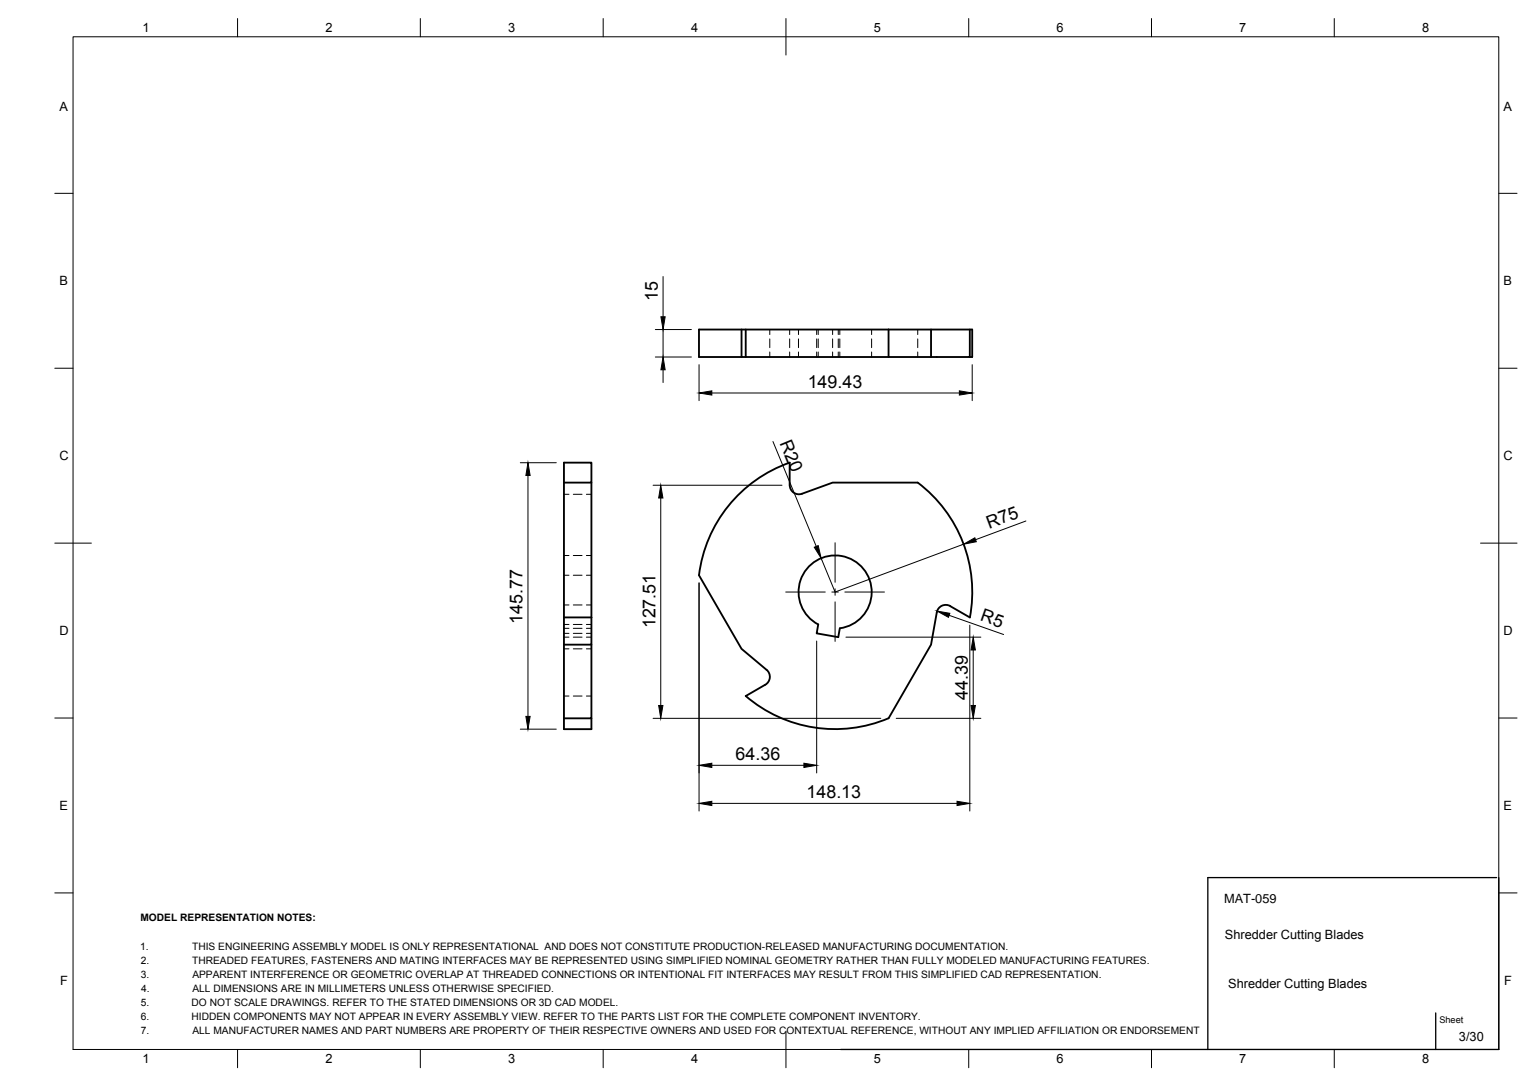
ISO-10303-21;
HEADER;
/* Generated by software containing ST-Developer
 * from STEP Tools, Inc. (www.steptools.com) 
 */

FILE_DESCRIPTION(
/* description */ ('', 'CAx-IF Rec.Pracs.---Representation and Presentation of Product Manufa
cturing Information (PMI)---4.0---2014-10-13'),
/* implementation_level */ '2;1');

FILE_NAME(
/* name */ 'Shredder Cutting Blades.step',
/* time_stamp */ '2026-10-28T23:00:48+01:00',
/* author */ (''),
/* organization */ (''),
/* preprocessor_version */ 'ST-DEVELOPER v20.2',
/* originating_system */ 'Autodesk Translation Framework v15.17.0.0',
/* authorisation */ '');

FILE_SCHEMA (('AP242_MANAGED_MODEL_BASED_3D_ENGINEERING_MIM_LF { 1 0 10303 442 2 1 4 }'));
ENDSEC;

DATA;
#10=MECHANICAL_DESIGN_GEOMETRIC_PRESENTATION_REPRESENTATION('',(#961),#61811);
#911=SHAPE_REPRESENTATION_RELATIONSHIP('SRR','None',#61969,#936);
#936=ADVANCED_BREP_SHAPE_REPRESENTATION('',(#1000),#61782);
#961=STYLED_ITEM('',(#62149),#1000);
#1000=MANIFOLD_SOLID_BREP('Body1',#33791);
#1038=CYLINDRICAL_SURFACE('',#34129,20.);
#1039=CYLINDRICAL_SURFACE('',#34132,5.);
#1040=CYLINDRICAL_SURFACE('',#34137,5.);
#1041=CYLINDRICAL_SURFACE('',#34141,75.);
#1042=CYLINDRICAL_SURFACE('',#34143,75.);
#1043=CYLINDRICAL_SURFACE('',#34145,5.);
#1044=CYLINDRICAL_SURFACE('',#34150,75.);
#1878=FACE_BOUND('',#6114,.T.);
#1879=FACE_BOUND('',#6132,.T.);
#2236=CIRCLE('',#34122,5.);
#2237=CIRCLE('',#34123,75.);
#2238=CIRCLE('',#34124,5.);
#2239=CIRCLE('',#34125,75.);
#2240=CIRCLE('',#34126,5.);
#2241=CIRCLE('',#34127,75.);
#2242=CIRCLE('',#34128,20.);
#2243=CIRCLE('',#34130,20.);
#2244=CIRCLE('',#34133,5.);
#2245=CIRCLE('',#34138,5.);
#2246=CIRCLE('',#34142,75.);
#2247=CIRCLE('',#34144,75.);
#2248=CIRCLE('',#34146,5.);
#2249=CIRCLE('',#34151,75.);
#4232=FACE_OUTER_BOUND('',#6110,.T.);
#4233=FACE_OUTER_BOUND('',#6111,.T.);
#4234=FACE_OUTER_BOUND('',#6112,.T.);
#4235=FACE_OUTER_BOUND('',#6113,.T.);
#4236=FACE_OUTER_BOUND('',#6115,.T.);
#4237=FACE_OUTER_BOUND('',#6116,.T.);
#4238=FACE_OUTER_BOUND('',#6117,.T.);
#4239=FACE_OUTER_BOUND('',#6118,.T.);
#4240=FACE_OUTER_BOUND('',#6119,.T.);
#4241=FACE_OUTER_BOUND('',#6120,.T.);
#4242=FACE_OUTER_BOUND('',#6121,.T.);
#4243=FACE_OUTER_BOUND('',#6122,.T.);
#4244=FACE_OUTER_BOUND('',#6123,.T.);
#4245=FACE_OUTER_BOUND('',#6124,.T.);
#4246=FACE_OUTER_BOUND('',#6125,.T.);
#4247=FACE_OUTER_BOUND('',#6126,.T.);
#4248=FACE_OUTER_BOUND('',#6127,.T.);
#4249=FACE_OUTER_BOUND('',#6128,.T.);
#4250=FACE_OUTER_BOUND('',#6129,.T.);
#4251=FACE_OUTER_BOUND('',#6130,.T.);
#4252=FACE_OUTER_BOUND('',#6131,.T.);
#6110=EDGE_LOOP('',(#21458,#21459,#21460,#21461));
#6111=EDGE_LOOP('',(#21462,#21463,#21464,#21465));
#6112=EDGE_LOOP('',(#21466,#21467,#21468,#21469));
#6113=EDGE_LOOP('',(#21470,#21471,#21472,#21473,#21474,#21475,#21476,#21477,
#21478,#21479,#21480,#21481,#21482,#21483,#21484));
#6114=EDGE_LOOP('',(#21485,#21486,#21487,#21488));
#6115=EDGE_LOOP('',(#21489,#21490,#21491,#21492));
#6116=EDGE_LOOP('',(#21493,#21494,#21495,#21496));
#6117=EDGE_LOOP('',(#21497,#21498,#21499,#21500));
#6118=EDGE_LOOP('',(#21501,#21502,#21503,#21504));
#6119=EDGE_LOOP('',(#21505,#21506,#21507,#21508));
#6120=EDGE_LOOP('',(#21509,#21510,#21511,#21512));
#6121=EDGE_LOOP('',(#21513,#21514,#21515,#21516));
#6122=EDGE_LOOP('',(#21517,#21518,#21519,#21520));
#6123=EDGE_LOOP('',(#21521,#21522,#21523,#21524));
#6124=EDGE_LOOP('',(#21525,#21526,#21527,#21528));
#6125=EDGE_LOOP('',(#21529,#21530,#21531,#21532));
#6126=EDGE_LOOP('',(#21533,#21534,#21535,#21536));
#6127=EDGE_LOOP('',(#21537,#21538,#21539,#21540));
#6128=EDGE_LOOP('',(#21541,#21542,#21543,#21544));
#6129=EDGE_LOOP('',(#21545,#21546,#21547,#21548));
#6130=EDGE_LOOP('',(#21549,#21550,#21551,#21552));
#6131=EDGE_LOOP('',(#21553,#21554,#21555,#21556,#21557,#21558,#21559,#21560,
#21561,#21562,#21563,#21564,#21565,#21566,#21567));
#6132=EDGE_LOOP('',(#21568,#21569,#21570,#21571));
#8346=LINE('',#48842,#10893);
#8347=LINE('',#48844,#10894);
#8348=LINE('',#48846,#10895);
#8349=LINE('',#48847,#10896);
#8350=LINE('',#48851,#10897);
#8351=LINE('',#48853,#10898);
#8352=LINE('',#48855,#10899);
#8353=LINE('',#48856,#10900);
#8354=LINE('',#48858,#10901);
#8355=LINE('',#48859,#10902);
#8356=LINE('',#48863,#10903);
#8357=LINE('',#48865,#10904);
#8358=LINE('',#48869,#10905);
#8359=LINE('',#48873,#10906);
#8360=LINE('',#48875,#10907);
#8361=LINE('',#48879,#10908);
#8362=LINE('',#48883,#10909);
#8363=LINE('',#48885,#10910);
#8364=LINE('',#48889,#10911);
#8365=LINE('',#48896,#10912);
#8366=LINE('',#48898,#10913);
#8367=LINE('',#48899,#10914);
#8368=LINE('',#48902,#10915);
#8369=LINE('',#48906,#10916);
#8370=LINE('',#48907,#10917);
#8371=LINE('',#48910,#10918);
#8372=LINE('',#48911,#10919);
#8373=LINE('',#48914,#10920);
#8374=LINE('',#48916,#10921);
#8375=LINE('',#48917,#10922);
#8376=LINE('',#48920,#10923);
#8377=LINE('',#48924,#10924);
#8378=LINE('',#48925,#10925);
#8379=LINE('',#48928,#10926);
#8380=LINE('',#48929,#10927);
#8381=LINE('',#48933,#10928);
#8382=LINE('',#48938,#10929);
#8383=LINE('',#48941,#10930);
#8384=LINE('',#48944,#10931);
#8385=LINE('',#48945,#10932);
#8386=LINE('',#48947,#10933);
#8387=LINE('',#48950,#10934);
#8388=LINE('',#48951,#10935);
#10893=VECTOR('',#38180,10.);
#10894=VECTOR('',#38181,10.);
#10895=VECTOR('',#38182,10.);
#10896=VECTOR('',#38183,10.);
#10897=VECTOR('',#38186,10.);
#10898=VECTOR('',#38187,10.);
#10899=VECTOR('',#38188,10.);
#10900=VECTOR('',#38189,10.);
#10901=VECTOR('',#38192,9.99999999999999);
#10902=VECTOR('',#38193,9.99999999999999);
#10903=VECTOR('',#38196,10.);
#10904=VECTOR('',#38197,9.99999999999999);
#10905=VECTOR('',#38200,10.);
#10906=VECTOR('',#38203,10.);
#10907=VECTOR('',#38204,10.);
#10908=VECTOR('',#38207,10.);
#10909=VECTOR('',#38210,10.);
#10910=VECTOR('',#38211,10.);
#10911=VECTOR('',#38214,10.);
#10912=VECTOR('',#38225,10.);
#10913=VECTOR('',#38226,10.);
#10914=VECTOR('',#38227,10.);
#10915=VECTOR('',#38230,10.);
#10916=VECTOR('',#38235,10.);
#10917=VECTOR('',#38236,9.99999999999999);
#10918=VECTOR('',#38239,10.);
#10919=VECTOR('',#38240,10.);
#10920=VECTOR('',#38243,10.);
#10921=VECTOR('',#38244,10.);
#10922=VECTOR('',#38245,10.);
#10923=VECTOR('',#38248,10.);
#10924=VECTOR('',#38253,10.);
#10925=VECTOR('',#38254,10.);
#10926=VECTOR('',#38257,10.);
#10927=VECTOR('',#38258,10.);
#10928=VECTOR('',#38263,10.);
#10929=VECTOR('',#38270,10.);
#10930=VECTOR('',#38273,10.);
#10931=VECTOR('',#38276,10.);
#10932=VECTOR('',#38277,10.);
#10933=VECTOR('',#38280,10.);
#10934=VECTOR('',#38283,10.);
#10935=VECTOR('',#38284,10.);
#13440=VERTEX_POINT('',#48840);
#13441=VERTEX_POINT('',#48841);
#13442=VERTEX_POINT('',#48843);
#13443=VERTEX_POINT('',#48845);
#13444=VERTEX_POINT('',#48849);
#13445=VERTEX_POINT('',#48850);
#13446=VERTEX_POINT('',#48852);
#13447=VERTEX_POINT('',#48854);
#13448=VERTEX_POINT('',#48861);
#13449=VERTEX_POINT('',#48862);
#13450=VERTEX_POINT('',#48864);
#13451=VERTEX_POINT('',#48866);
#13452=VERTEX_POINT('',#48868);
#13453=VERTEX_POINT('',#48870);
#13454=VERTEX_POINT('',#48872);
#13455=VERTEX_POINT('',#48874);
#13456=VERTEX_POINT('',#48876);
#13457=VERTEX_POINT('',#48878);
#13458=VERTEX_POINT('',#48880);
#13459=VERTEX_POINT('',#48882);
#13460=VERTEX_POINT('',#48884);
#13461=VERTEX_POINT('',#48886);
#13462=VERTEX_POINT('',#48888);
#13463=VERTEX_POINT('',#48895);
#13464=VERTEX_POINT('',#48897);
#13465=VERTEX_POINT('',#48901);
#13466=VERTEX_POINT('',#48905);
#13467=VERTEX_POINT('',#48909);
#13468=VERTEX_POINT('',#48913);
#13469=VERTEX_POINT('',#48915);
#13470=VERTEX_POINT('',#48919);
#13471=VERTEX_POINT('',#48923);
#13472=VERTEX_POINT('',#48927);
#13473=VERTEX_POINT('',#48931);
#13474=VERTEX_POINT('',#48937);
#13475=VERTEX_POINT('',#48939);
#13476=VERTEX_POINT('',#48943);
#13477=VERTEX_POINT('',#48949);
#16631=EDGE_CURVE('',#13440,#13441,#8346,.T.);
#16632=EDGE_CURVE('',#13440,#13442,#8347,.T.);
#16633=EDGE_CURVE('',#13443,#13442,#8348,.T.);
#16634=EDGE_CURVE('',#13441,#13443,#8349,.T.);
#16635=EDGE_CURVE('',#13444,#13445,#8350,.T.);
#16636=EDGE_CURVE('',#13446,#13444,#8351,.T.);
#16637=EDGE_CURVE('',#13447,#13446,#8352,.T.);
#16638=EDGE_CURVE('',#13445,#13447,#8353,.T.);
#16639=EDGE_CURVE('',#13445,#13440,#8354,.T.);
#16640=EDGE_CURVE('',#13442,#13447,#8355,.T.);
#16641=EDGE_CURVE('',#13448,#13449,#8356,.T.);
#16642=EDGE_CURVE('',#13449,#13450,#8357,.T.);
#16643=EDGE_CURVE('',#13450,#13451,#2236,.T.);
#16644=EDGE_CURVE('',#13451,#13452,#8358,.T.);
#16645=EDGE_CURVE('',#13453,#13452,#2237,.T.);
#16646=EDGE_CURVE('',#13453,#13454,#8359,.T.);
#16647=EDGE_CURVE('',#13454,#13455,#8360,.T.);
#16648=EDGE_CURVE('',#13455,#13456,#2238,.T.);
#16649=EDGE_CURVE('',#13456,#13457,#8361,.T.);
#16650=EDGE_CURVE('',#13458,#13457,#2239,.T.);
#16651=EDGE_CURVE('',#13458,#13459,#8362,.T.);
#16652=EDGE_CURVE('',#13459,#13460,#8363,.T.);
#16653=EDGE_CURVE('',#13460,#13461,#2240,.T.);
#16654=EDGE_CURVE('',#13461,#13462,#8364,.T.);
#16655=EDGE_CURVE('',#13448,#13462,#2241,.T.);
#16656=EDGE_CURVE('',#13446,#13443,#2242,.T.);
#16657=EDGE_CURVE('',#13441,#13444,#2243,.T.);
#16658=EDGE_CURVE('',#13452,#13463,#8365,.T.);
#16659=EDGE_CURVE('',#13451,#13464,#8366,.T.);
#16660=EDGE_CURVE('',#13463,#13464,#8367,.T.);
#16661=EDGE_CURVE('',#13450,#13465,#8368,.T.);
#16662=EDGE_CURVE('',#13464,#13465,#2244,.T.);
#16663=EDGE_CURVE('',#13449,#13466,#8369,.T.);
#16664=EDGE_CURVE('',#13465,#13466,#8370,.T.);
#16665=EDGE_CURVE('',#13467,#13448,#8371,.T.);
#16666=EDGE_CURVE('',#13466,#13467,#8372,.T.);
#16667=EDGE_CURVE('',#13457,#13468,#8373,.T.);
#16668=EDGE_CURVE('',#13456,#13469,#8374,.T.);
#16669=EDGE_CURVE('',#13468,#13469,#8375,.T.);
#16670=EDGE_CURVE('',#13455,#13470,#8376,.T.);
#16671=EDGE_CURVE('',#13469,#13470,#2245,.T.);
#16672=EDGE_CURVE('',#13454,#13471,#8377,.T.);
#16673=EDGE_CURVE('',#13470,#13471,#8378,.T.);
#16674=EDGE_CURVE('',#13472,#13453,#8379,.T.);
#16675=EDGE_CURVE('',#13471,#13472,#8380,.T.);
#16676=EDGE_CURVE('',#13473,#13468,#2246,.T.);
#16677=EDGE_CURVE('',#13473,#13458,#8381,.T.);
#16678=EDGE_CURVE('',#13472,#13463,#2247,.T.);
#16679=EDGE_CURVE('',#13460,#13474,#8382,.T.);
#16680=EDGE_CURVE('',#13475,#13474,#2248,.T.);
#16681=EDGE_CURVE('',#13461,#13475,#8383,.T.);
#16682=EDGE_CURVE('',#13459,#13476,#8384,.T.);
#16683=EDGE_CURVE('',#13474,#13476,#8385,.T.);
#16684=EDGE_CURVE('',#13476,#13473,#8386,.T.);
#16685=EDGE_CURVE('',#13462,#13477,#8387,.T.);
#16686=EDGE_CURVE('',#13477,#13475,#8388,.T.);
#16687=EDGE_CURVE('',#13467,#13477,#2249,.T.);
#21458=ORIENTED_EDGE('',*,*,#16631,.F.);
#21459=ORIENTED_EDGE('',*,*,#16632,.T.);
#21460=ORIENTED_EDGE('',*,*,#16633,.F.);
#21461=ORIENTED_EDGE('',*,*,#16634,.F.);
#21462=ORIENTED_EDGE('',*,*,#16635,.F.);
#21463=ORIENTED_EDGE('',*,*,#16636,.F.);
#21464=ORIENTED_EDGE('',*,*,#16637,.F.);
#21465=ORIENTED_EDGE('',*,*,#16638,.F.);
#21466=ORIENTED_EDGE('',*,*,#16639,.F.);
#21467=ORIENTED_EDGE('',*,*,#16638,.T.);
#21468=ORIENTED_EDGE('',*,*,#16640,.F.);
#21469=ORIENTED_EDGE('',*,*,#16632,.F.);
#21470=ORIENTED_EDGE('',*,*,#16641,.T.);
#21471=ORIENTED_EDGE('',*,*,#16642,.T.);
#21472=ORIENTED_EDGE('',*,*,#16643,.T.);
#21473=ORIENTED_EDGE('',*,*,#16644,.T.);
#21474=ORIENTED_EDGE('',*,*,#16645,.F.);
#21475=ORIENTED_EDGE('',*,*,#16646,.T.);
#21476=ORIENTED_EDGE('',*,*,#16647,.T.);
#21477=ORIENTED_EDGE('',*,*,#16648,.T.);
#21478=ORIENTED_EDGE('',*,*,#16649,.T.);
#21479=ORIENTED_EDGE('',*,*,#16650,.F.);
#21480=ORIENTED_EDGE('',*,*,#16651,.T.);
#21481=ORIENTED_EDGE('',*,*,#16652,.T.);
#21482=ORIENTED_EDGE('',*,*,#16653,.T.);
#21483=ORIENTED_EDGE('',*,*,#16654,.T.);
#21484=ORIENTED_EDGE('',*,*,#16655,.F.);
#21485=ORIENTED_EDGE('',*,*,#16633,.T.);
#21486=ORIENTED_EDGE('',*,*,#16640,.T.);
#21487=ORIENTED_EDGE('',*,*,#16637,.T.);
#21488=ORIENTED_EDGE('',*,*,#16656,.T.);
#21489=ORIENTED_EDGE('',*,*,#16634,.T.);
#21490=ORIENTED_EDGE('',*,*,#16656,.F.);
#21491=ORIENTED_EDGE('',*,*,#16636,.T.);
#21492=ORIENTED_EDGE('',*,*,#16657,.F.);
#21493=ORIENTED_EDGE('',*,*,#16658,.F.);
#21494=ORIENTED_EDGE('',*,*,#16644,.F.);
#21495=ORIENTED_EDGE('',*,*,#16659,.T.);
#21496=ORIENTED_EDGE('',*,*,#16660,.F.);
#21497=ORIENTED_EDGE('',*,*,#16643,.F.);
#21498=ORIENTED_EDGE('',*,*,#16661,.T.);
#21499=ORIENTED_EDGE('',*,*,#16662,.F.);
#21500=ORIENTED_EDGE('',*,*,#16659,.F.);
#21501=ORIENTED_EDGE('',*,*,#16642,.F.);
#21502=ORIENTED_EDGE('',*,*,#16663,.T.);
#21503=ORIENTED_EDGE('',*,*,#16664,.F.);
#21504=ORIENTED_EDGE('',*,*,#16661,.F.);
#21505=ORIENTED_EDGE('',*,*,#16665,.F.);
#21506=ORIENTED_EDGE('',*,*,#16666,.F.);
#21507=ORIENTED_EDGE('',*,*,#16663,.F.);
#21508=ORIENTED_EDGE('',*,*,#16641,.F.);
#21509=ORIENTED_EDGE('',*,*,#16667,.F.);
#21510=ORIENTED_EDGE('',*,*,#16649,.F.);
#21511=ORIENTED_EDGE('',*,*,#16668,.T.);
#21512=ORIENTED_EDGE('',*,*,#16669,.F.);
#21513=ORIENTED_EDGE('',*,*,#16648,.F.);
#21514=ORIENTED_EDGE('',*,*,#16670,.T.);
#21515=ORIENTED_EDGE('',*,*,#16671,.F.);
#21516=ORIENTED_EDGE('',*,*,#16668,.F.);
#21517=ORIENTED_EDGE('',*,*,#16647,.F.);
#21518=ORIENTED_EDGE('',*,*,#16672,.T.);
#21519=ORIENTED_EDGE('',*,*,#16673,.F.);
#21520=ORIENTED_EDGE('',*,*,#16670,.F.);
#21521=ORIENTED_EDGE('',*,*,#16674,.F.);
#21522=ORIENTED_EDGE('',*,*,#16675,.F.);
#21523=ORIENTED_EDGE('',*,*,#16672,.F.);
#21524=ORIENTED_EDGE('',*,*,#16646,.F.);
#21525=ORIENTED_EDGE('',*,*,#16667,.T.);
#21526=ORIENTED_EDGE('',*,*,#16676,.F.);
#21527=ORIENTED_EDGE('',*,*,#16677,.T.);
#21528=ORIENTED_EDGE('',*,*,#16650,.T.);
#21529=ORIENTED_EDGE('',*,*,#16658,.T.);
#21530=ORIENTED_EDGE('',*,*,#16678,.F.);
#21531=ORIENTED_EDGE('',*,*,#16674,.T.);
#21532=ORIENTED_EDGE('',*,*,#16645,.T.);
#21533=ORIENTED_EDGE('',*,*,#16653,.F.);
#21534=ORIENTED_EDGE('',*,*,#16679,.T.);
#21535=ORIENTED_EDGE('',*,*,#16680,.F.);
#21536=ORIENTED_EDGE('',*,*,#16681,.F.);
#21537=ORIENTED_EDGE('',*,*,#16652,.F.);
#21538=ORIENTED_EDGE('',*,*,#16682,.T.);
#21539=ORIENTED_EDGE('',*,*,#16683,.F.);
#21540=ORIENTED_EDGE('',*,*,#16679,.F.);
#21541=ORIENTED_EDGE('',*,*,#16677,.F.);
#21542=ORIENTED_EDGE('',*,*,#16684,.F.);
#21543=ORIENTED_EDGE('',*,*,#16682,.F.);
#21544=ORIENTED_EDGE('',*,*,#16651,.F.);
#21545=ORIENTED_EDGE('',*,*,#16685,.F.);
#21546=ORIENTED_EDGE('',*,*,#16654,.F.);
#21547=ORIENTED_EDGE('',*,*,#16681,.T.);
#21548=ORIENTED_EDGE('',*,*,#16686,.F.);
#21549=ORIENTED_EDGE('',*,*,#16665,.T.);
#21550=ORIENTED_EDGE('',*,*,#16655,.T.);
#21551=ORIENTED_EDGE('',*,*,#16685,.T.);
#21552=ORIENTED_EDGE('',*,*,#16687,.F.);
#21553=ORIENTED_EDGE('',*,*,#16666,.T.);
#21554=ORIENTED_EDGE('',*,*,#16687,.T.);
#21555=ORIENTED_EDGE('',*,*,#16686,.T.);
#21556=ORIENTED_EDGE('',*,*,#16680,.T.);
#21557=ORIENTED_EDGE('',*,*,#16683,.T.);
#21558=ORIENTED_EDGE('',*,*,#16684,.T.);
#21559=ORIENTED_EDGE('',*,*,#16676,.T.);
#21560=ORIENTED_EDGE('',*,*,#16669,.T.);
#21561=ORIENTED_EDGE('',*,*,#16671,.T.);
#21562=ORIENTED_EDGE('',*,*,#16673,.T.);
#21563=ORIENTED_EDGE('',*,*,#16675,.T.);
#21564=ORIENTED_EDGE('',*,*,#16678,.T.);
#21565=ORIENTED_EDGE('',*,*,#16660,.T.);
#21566=ORIENTED_EDGE('',*,*,#16662,.T.);
#21567=ORIENTED_EDGE('',*,*,#16664,.T.);
#21568=ORIENTED_EDGE('',*,*,#16631,.T.);
#21569=ORIENTED_EDGE('',*,*,#16657,.T.);
#21570=ORIENTED_EDGE('',*,*,#16635,.T.);
#21571=ORIENTED_EDGE('',*,*,#16639,.T.);
#31112=PLANE('',#34118);
#31113=PLANE('',#34119);
#31114=PLANE('',#34120);
#31115=PLANE('',#34121);
#31116=PLANE('',#34131);
#31117=PLANE('',#34134);
#31118=PLANE('',#34135);
#31119=PLANE('',#34136);
#31120=PLANE('',#34139);
#31121=PLANE('',#34140);
#31122=PLANE('',#34147);
#31123=PLANE('',#34148);
#31124=PLANE('',#34149);
#31125=PLANE('',#34152);
#31913=ADVANCED_FACE('',(#4232),#31112,.F.);
#31914=ADVANCED_FACE('',(#4233),#31113,.F.);
#31915=ADVANCED_FACE('',(#4234),#31114,.F.);
#31916=ADVANCED_FACE('',(#4235,#1878),#31115,.F.);
#31917=ADVANCED_FACE('',(#4236),#1038,.F.);
#31918=ADVANCED_FACE('',(#4237),#31116,.F.);
#31919=ADVANCED_FACE('',(#4238),#1039,.F.);
#31920=ADVANCED_FACE('',(#4239),#31117,.F.);
#31921=ADVANCED_FACE('',(#4240),#31118,.F.);
#31922=ADVANCED_FACE('',(#4241),#31119,.F.);
#31923=ADVANCED_FACE('',(#4242),#1040,.F.);
#31924=ADVANCED_FACE('',(#4243),#31120,.F.);
#31925=ADVANCED_FACE('',(#4244),#31121,.F.);
#31926=ADVANCED_FACE('',(#4245),#1041,.T.);
#31927=ADVANCED_FACE('',(#4246),#1042,.T.);
#31928=ADVANCED_FACE('',(#4247),#1043,.F.);
#31929=ADVANCED_FACE('',(#4248),#31122,.F.);
#31930=ADVANCED_FACE('',(#4249),#31123,.F.);
#31931=ADVANCED_FACE('',(#4250),#31124,.F.);
#31932=ADVANCED_FACE('',(#4251),#1044,.T.);
#31933=ADVANCED_FACE('',(#4252,#1879),#31125,.T.);
#33791=CLOSED_SHELL('',(#31913,#31914,#31915,#31916,#31917,#31918,#31919,
#31920,#31921,#31922,#31923,#31924,#31925,#31926,#31927,#31928,#31929,#31930,
#31931,#31932,#31933));
#34117=AXIS2_PLACEMENT_3D('',#48838,#38176,#38177);
#34118=AXIS2_PLACEMENT_3D('',#48839,#38178,#38179);
#34119=AXIS2_PLACEMENT_3D('',#48848,#38184,#38185);
#34120=AXIS2_PLACEMENT_3D('',#48857,#38190,#38191);
#34121=AXIS2_PLACEMENT_3D('',#48860,#38194,#38195);
#34122=AXIS2_PLACEMENT_3D('',#48867,#38198,#38199);
#34123=AXIS2_PLACEMENT_3D('',#48871,#38201,#38202);
#34124=AXIS2_PLACEMENT_3D('',#48877,#38205,#38206);
#34125=AXIS2_PLACEMENT_3D('',#48881,#38208,#38209);
#34126=AXIS2_PLACEMENT_3D('',#48887,#38212,#38213);
#34127=AXIS2_PLACEMENT_3D('',#48890,#38215,#38216);
#34128=AXIS2_PLACEMENT_3D('',#48891,#38217,#38218);
#34129=AXIS2_PLACEMENT_3D('',#48892,#38219,#38220);
#34130=AXIS2_PLACEMENT_3D('',#48893,#38221,#38222);
#34131=AXIS2_PLACEMENT_3D('',#48894,#38223,#38224);
#34132=AXIS2_PLACEMENT_3D('',#48900,#38228,#38229);
#34133=AXIS2_PLACEMENT_3D('',#48903,#38231,#38232);
#34134=AXIS2_PLACEMENT_3D('',#48904,#38233,#38234);
#34135=AXIS2_PLACEMENT_3D('',#48908,#38237,#38238);
#34136=AXIS2_PLACEMENT_3D('',#48912,#38241,#38242);
#34137=AXIS2_PLACEMENT_3D('',#48918,#38246,#38247);
#34138=AXIS2_PLACEMENT_3D('',#48921,#38249,#38250);
#34139=AXIS2_PLACEMENT_3D('',#48922,#38251,#38252);
#34140=AXIS2_PLACEMENT_3D('',#48926,#38255,#38256);
#34141=AXIS2_PLACEMENT_3D('',#48930,#38259,#38260);
#34142=AXIS2_PLACEMENT_3D('',#48932,#38261,#38262);
#34143=AXIS2_PLACEMENT_3D('',#48934,#38264,#38265);
#34144=AXIS2_PLACEMENT_3D('',#48935,#38266,#38267);
#34145=AXIS2_PLACEMENT_3D('',#48936,#38268,#38269);
#34146=AXIS2_PLACEMENT_3D('',#48940,#38271,#38272);
#34147=AXIS2_PLACEMENT_3D('',#48942,#38274,#38275);
#34148=AXIS2_PLACEMENT_3D('',#48946,#38278,#38279);
#34149=AXIS2_PLACEMENT_3D('',#48948,#38281,#38282);
#34150=AXIS2_PLACEMENT_3D('',#48952,#38285,#38286);
#34151=AXIS2_PLACEMENT_3D('',#48953,#38287,#38288);
#34152=AXIS2_PLACEMENT_3D('',#48954,#38289,#38290);
#38176=DIRECTION('axis',(0.,0.,1.));
#38177=DIRECTION('refdir',(1.,0.,0.));
#38178=DIRECTION('center_axis',(0.996957691137886,-6.79465961587148E-16,
0.077944609056791));
#38179=DIRECTION('ref_axis',(0.077944609056791,2.83369376080442E-15,-0.996957691137886));
#38180=DIRECTION('',(-0.077944609056791,-2.83369376080442E-15,0.996957691137886));
#38181=DIRECTION('',(-4.56527663898138E-16,-1.,-2.87803349790671E-15));
#38182=DIRECTION('',(0.077944609056791,2.83369376080442E-15,-0.996957691137886));
#38183=DIRECTION('',(-4.56527663898138E-16,-1.,-2.87803349790671E-15));
#38184=DIRECTION('center_axis',(-0.996957691137886,6.79465961587148E-16,
-0.077944609056791));
#38185=DIRECTION('ref_axis',(-0.077944609056791,-2.83369376080442E-15,0.996957691137886));
#38186=DIRECTION('',(0.077944609056791,2.83369376080442E-15,-0.996957691137886));
#38187=DIRECTION('',(4.56527663898138E-16,1.,2.87803349790671E-15));
#38188=DIRECTION('',(-0.077944609056791,-2.83369376080442E-15,0.996957691137886));
#38189=DIRECTION('',(-4.56527663898138E-16,-1.,-2.87803349790671E-15));
#38190=DIRECTION('center_axis',(0.0779446090567893,2.83369376080442E-15,
-0.996957691137886));
#38191=DIRECTION('ref_axis',(-0.996957691137886,6.79465961587143E-16,-0.0779446090567894));
#38192=DIRECTION('',(0.996957691137886,-6.79465961587143E-16,0.0779446090567893));
#38193=DIRECTION('',(-0.996957691137886,6.79465961587143E-16,-0.0779446090567893));
#38194=DIRECTION('center_axis',(4.56527663898138E-16,1.,2.87803349790671E-15));
#38195=DIRECTION('ref_axis',(0.902362991552081,8.2841209666094E-16,-0.430976834037722));
#38196=DIRECTION('',(0.267735638451905,-2.89519216216193E-15,0.963492411959093));
#38197=DIRECTION('',(-0.0779446090567835,-2.83369376080443E-15,0.996957691137886));
#38198=DIRECTION('center_axis',(4.56527663898138E-16,1.,2.87803349790671E-15));
#38199=DIRECTION('ref_axis',(0.267735638451906,-2.89519216216193E-15,0.963492411959093));
#38200=DIRECTION('',(0.963492411959093,3.30691196032757E-16,-0.267735638451905));
#38201=DIRECTION('center_axis',(4.56527663898138E-16,1.,2.87803349790671E-15));
#38202=DIRECTION('ref_axis',(0.902362991552081,8.2841209666094E-16,-0.430976834037722));
#38203=DIRECTION('',(-0.968276724336069,1.16120910450874E-15,-0.249880341581751));
#38204=DIRECTION('',(-0.824418382495298,2.00528166414349E-15,-0.565980857100164));
#38205=DIRECTION('center_axis',(4.56527663898138E-16,1.,2.87803349790671E-15));
#38206=DIRECTION('ref_axis',(-0.968276724336069,1.16120910450873E-15,-0.24988034158175));
#38207=DIRECTION('',(-0.249880341581751,-2.67265555928621E-15,0.968276724336069));
#38208=DIRECTION('center_axis',(4.56527663898138E-16,1.,2.87803349790671E-15));
#38209=DIRECTION('ref_axis',(0.902362991552081,8.2841209666094E-16,-0.430976834037722));
#38210=DIRECTION('',(0.700541085884164,1.73398305765319E-15,-0.713612070377342));
#38211=DIRECTION('',(0.902362991552081,8.2841209666094E-16,-0.430976834037722));
#38212=DIRECTION('center_axis',(4.56527663898138E-16,1.,2.87803349790671E-15));
#38213=DIRECTION('ref_axis',(0.700541085884163,1.73398305765319E-15,-0.713612070377343));
#38214=DIRECTION('',(-0.713612070377342,2.34196436325345E-15,-0.700541085884164));
#38215=DIRECTION('center_axis',(4.56527663898138E-16,1.,2.87803349790671E-15));
#38216=DIRECTION('ref_axis',(0.902362991552081,8.2841209666094E-16,-0.430976834037722));
#38217=DIRECTION('center_axis',(4.56527663898138E-16,1.,2.87803349790671E-15));
#38218=DIRECTION('ref_axis',(-0.902362991552081,-8.2841209666094E-16,0.430976834037722));
#38219=DIRECTION('center_axis',(4.56527663898138E-16,1.,2.87803349790671E-15));
#38220=DIRECTION('ref_axis',(-0.0779446090567806,-2.83369376080443E-15,
0.996957691137887));
#38221=DIRECTION('center_axis',(-4.56527663898138E-16,-1.,-2.87803349790671E-15));
#38222=DIRECTION('ref_axis',(-0.902362991552081,-8.2841209666094E-16,0.430976834037722));
#38223=DIRECTION('center_axis',(0.267735638451905,-2.89519216216193E-15,
0.963492411959093));
#38224=DIRECTION('ref_axis',(0.963492411959093,3.30691196032758E-16,-0.267735638451905));
#38225=DIRECTION('',(4.56527663898138E-16,1.,2.87803349790671E-15));
#38226=DIRECTION('',(4.56527663898138E-16,1.,2.87803349790671E-15));
#38227=DIRECTION('',(-0.963492411959093,-3.30691196032757E-16,0.267735638451905));
#38228=DIRECTION('center_axis',(4.56527663898138E-16,1.,2.87803349790671E-15));
#38229=DIRECTION('ref_axis',(0.267735638451906,-2.89519216216193E-15,0.963492411959093));
#38230=DIRECTION('',(4.56527663898138E-16,1.,2.87803349790671E-15));
#38231=DIRECTION('center_axis',(-4.56527663898138E-16,-1.,-2.87803349790671E-15));
#38232=DIRECTION('ref_axis',(0.267735638451906,-2.89519216216193E-15,0.963492411959093));
#38233=DIRECTION('center_axis',(-0.996957691137886,6.79465961587129E-16,
-0.0779446090567844));
#38234=DIRECTION('ref_axis',(-0.0779446090567843,-2.83369376080442E-15,
0.996957691137886));
#38235=DIRECTION('',(4.56527663898138E-16,1.,2.87803349790671E-15));
#38236=DIRECTION('',(0.0779446090567835,2.83369376080443E-15,-0.996957691137886));
#38237=DIRECTION('center_axis',(-0.963492411959093,-3.30691196032757E-16,
0.267735638451905));
#38238=DIRECTION('ref_axis',(0.267735638451905,-2.89519216216193E-15,0.963492411959093));
#38239=DIRECTION('',(-4.56527663898138E-16,-1.,-2.87803349790671E-15));
#38240=DIRECTION('',(-0.267735638451905,2.89519216216193E-15,-0.963492411959093));
#38241=DIRECTION('center_axis',(-0.968276724336069,1.16120910450874E-15,
-0.249880341581751));
#38242=DIRECTION('ref_axis',(-0.24988034158175,-2.67265555928621E-15,0.968276724336069));
#38243=DIRECTION('',(4.56527663898138E-16,1.,2.87803349790671E-15));
#38244=DIRECTION('',(4.56527663898138E-16,1.,2.87803349790671E-15));
#38245=DIRECTION('',(0.249880341581751,2.67265555928621E-15,-0.968276724336069));
#38246=DIRECTION('center_axis',(4.56527663898138E-16,1.,2.87803349790671E-15));
#38247=DIRECTION('ref_axis',(-0.968276724336069,1.16120910450873E-15,-0.24988034158175));
#38248=DIRECTION('',(4.56527663898138E-16,1.,2.87803349790671E-15));
#38249=DIRECTION('center_axis',(-4.56527663898138E-16,-1.,-2.87803349790671E-15));
#38250=DIRECTION('ref_axis',(-0.968276724336069,1.16120910450873E-15,-0.24988034158175));
#38251=DIRECTION('center_axis',(0.565980857100164,2.11431780260853E-15,
-0.824418382495298));
#38252=DIRECTION('ref_axis',(-0.824418382495298,2.00528166414349E-15,-0.565980857100164));
#38253=DIRECTION('',(4.56527663898138E-16,1.,2.87803349790671E-15));
#38254=DIRECTION('',(0.824418382495298,-2.00528166414349E-15,0.565980857100164));
#38255=DIRECTION('center_axis',(0.249880341581751,2.67265555928621E-15,
-0.968276724336069));
#38256=DIRECTION('ref_axis',(-0.968276724336069,1.16120910450874E-15,-0.24988034158175));
#38257=DIRECTION('',(-4.56527663898138E-16,-1.,-2.87803349790671E-15));
#38258=DIRECTION('',(0.968276724336069,-1.16120910450874E-15,0.249880341581751));
#38259=DIRECTION('center_axis',(4.56527663898138E-16,1.,2.87803349790671E-15));
#38260=DIRECTION('ref_axis',(-0.910727040524933,-7.72881033974921E-16,0.413008786415856));
#38261=DIRECTION('center_axis',(4.56527663898138E-16,1.,2.87803349790671E-15));
#38262=DIRECTION('ref_axis',(0.902362991552081,8.2841209666094E-16,-0.430976834037722));
#38263=DIRECTION('',(-4.56527663898138E-16,-1.,-2.87803349790671E-15));
#38264=DIRECTION('center_axis',(4.56527663898138E-16,1.,2.87803349790671E-15));
#38265=DIRECTION('ref_axis',(0.902362991552081,8.2841209666094E-16,-0.430976834037722));
#38266=DIRECTION('center_axis',(4.56527663898138E-16,1.,2.87803349790671E-15));
#38267=DIRECTION('ref_axis',(0.902362991552081,8.2841209666094E-16,-0.430976834037722));
#38268=DIRECTION('center_axis',(4.56527663898138E-16,1.,2.87803349790671E-15));
#38269=DIRECTION('ref_axis',(0.700541085884163,1.73398305765319E-15,-0.713612070377343));
#38270=DIRECTION('',(4.56527663898138E-16,1.,2.87803349790671E-15));
#38271=DIRECTION('center_axis',(-4.56527663898138E-16,-1.,-2.87803349790671E-15));
#38272=DIRECTION('ref_axis',(0.700541085884163,1.73398305765319E-15,-0.713612070377343));
#38273=DIRECTION('',(4.56527663898138E-16,1.,2.87803349790671E-15));
#38274=DIRECTION('center_axis',(0.430976834037722,-2.79378376419566E-15,
0.902362991552081));
#38275=DIRECTION('ref_axis',(0.902362991552081,8.2841209666094E-16,-0.430976834037722));
#38276=DIRECTION('',(4.56527663898138E-16,1.,2.87803349790671E-15));
#38277=DIRECTION('',(-0.902362991552081,-8.2841209666094E-16,0.430976834037722));
#38278=DIRECTION('center_axis',(0.713612070377342,-2.34196436325345E-15,
0.700541085884164));
#38279=DIRECTION('ref_axis',(0.700541085884164,1.73398305765319E-15,-0.713612070377342));
#38280=DIRECTION('',(-0.700541085884164,-1.73398305765319E-15,0.713612070377342));
#38281=DIRECTION('center_axis',(0.700541085884164,1.73398305765319E-15,
-0.713612070377342));
#38282=DIRECTION('ref_axis',(-0.713612070377342,2.34196436325345E-15,-0.700541085884164));
#38283=DIRECTION('',(4.56527663898138E-16,1.,2.87803349790671E-15));
#38284=DIRECTION('',(0.713612070377342,-2.34196436325345E-15,0.700541085884164));
#38285=DIRECTION('center_axis',(4.56527663898138E-16,1.,2.87803349790671E-15));
#38286=DIRECTION('ref_axis',(0.902362991552081,8.2841209666094E-16,-0.430976834037722));
#38287=DIRECTION('center_axis',(4.56527663898138E-16,1.,2.87803349790671E-15));
#38288=DIRECTION('ref_axis',(0.902362991552081,8.2841209666094E-16,-0.430976834037722));
#38289=DIRECTION('center_axis',(4.56527663898138E-16,1.,2.87803349790671E-15));
#38290=DIRECTION('ref_axis',(0.902362991552081,8.2841209666094E-16,-0.430976834037722));
#48838=CARTESIAN_POINT('',(0.,0.,0.));
#48839=CARTESIAN_POINT('Origin',(382.3447776627,-195.47200726879,429.516345148026));
#48840=CARTESIAN_POINT('',(382.968334535155,-195.47200726879,421.540683618923));
#48841=CARTESIAN_POINT('',(382.584752280159,-195.47200726879,426.446927731621));
#48842=CARTESIAN_POINT('',(382.937109532866,-195.47200726879,421.940069882636));
#48843=CARTESIAN_POINT('',(382.968334535155,-210.47200726879,421.540683618923));
#48844=CARTESIAN_POINT('',(382.968334535155,-195.47200726879,421.540683618923));
#48845=CARTESIAN_POINT('',(382.584752280159,-210.47200726879,426.446927731621));
#48846=CARTESIAN_POINT('',(382.937109532866,-210.47200726879,421.940069882636));
#48847=CARTESIAN_POINT('',(382.584752280159,-210.47200726879,426.446927731621));
#48848=CARTESIAN_POINT('Origin',(371.0048422415,-195.47200726879,420.605348310242));
#48849=CARTESIAN_POINT('',(370.621259986505,-195.47200726879,425.51159242294));
#48850=CARTESIAN_POINT('',(371.0048422415,-195.47200726879,420.605348310242));
#48851=CARTESIAN_POINT('',(371.285395675438,-195.47200726879,417.016903809402));
#48852=CARTESIAN_POINT('',(370.621259986505,-210.47200726879,425.51159242294));
#48853=CARTESIAN_POINT('',(370.621259986505,-210.47200726879,425.51159242294));
#48854=CARTESIAN_POINT('',(371.0048422415,-210.47200726879,420.605348310242));
#48855=CARTESIAN_POINT('',(371.285395675438,-210.47200726879,417.016903809402));
#48856=CARTESIAN_POINT('',(371.0048422415,-195.47200726879,420.605348310242));
#48857=CARTESIAN_POINT('Origin',(382.968334535155,-195.47200726879,421.540683618923));
#48858=CARTESIAN_POINT('',(353.029152922466,-195.47200726879,419.199964622495));
#48859=CARTESIAN_POINT('',(353.029152922466,-210.47200726879,419.199964622495));
#48860=CARTESIAN_POINT('Origin',(323.651078177653,-210.47200726879,409.682356624389));
#48861=CARTESIAN_POINT('',(420.687969084835,-210.47200726879,385.433330852756));
#48862=CARTESIAN_POINT('',(433.14196495934,-210.47200726879,430.251161579503));
#48863=CARTESIAN_POINT('',(420.081814582884,-210.47200726879,383.251980374045));
#48864=CARTESIAN_POINT('',(431.749931923224,-210.47200726879,448.056088160926));
#48865=CARTESIAN_POINT('',(433.608541542394,-210.47200726879,424.283370880314));
#48866=CARTESIAN_POINT('',(438.073398571173,-210.47200726879,453.263273266005));
#48867=CARTESIAN_POINT('Origin',(436.734720378913,-210.47200726879,448.44581120621));
#48868=CARTESIAN_POINT('',(449.951557303507,-210.47200726879,449.962565992797));
#48869=CARTESIAN_POINT('',(390.584364046299,-210.47200726879,466.459544269457));
#48870=CARTESIAN_POINT('',(403.916141292317,-210.47200726879,514.24988954184));
#48871=CARTESIAN_POINT('Origin',(375.115917770964,-210.47200726879,445.000000551892));
#48872=CARTESIAN_POINT('',(358.875763403191,-210.47200726879,502.626450984414));
#48873=CARTESIAN_POINT('',(354.564704687327,-210.47200726879,501.513908673498));
#48874=CARTESIAN_POINT('',(344.15226118922,-210.47200726879,492.518451721519));
#48875=CARTESIAN_POINT('',(325.221168140732,-210.47200726879,479.521851333988));
#48876=CARTESIAN_POINT('',(336.480973282039,-210.47200726879,495.391141926086));
#48877=CARTESIAN_POINT('Origin',(341.322356903719,-210.47200726879,496.640543633995));
#48878=CARTESIAN_POINT('',(333.400390264926,-210.47200726879,507.328282775076));
#48879=CARTESIAN_POINT('',(346.449185288851,-210.47200726879,456.764703334135));
#48880=CARTESIAN_POINT('',(300.743642935741,-210.47200726879,435.316781261079));
#48881=CARTESIAN_POINT('Origin',(375.115917770964,-210.47200726879,445.000000551892));
#48882=CARTESIAN_POINT('',(333.330024950362,-210.47200726879,402.122389091758));
#48883=CARTESIAN_POINT('',(312.102604347699,-210.47200726879,423.745879662505));
#48884=CARTESIAN_POINT('',(349.445560200449,-210.47200726879,394.42546177323));
#48885=CARTESIAN_POINT('',(327.919413934783,-210.47200726879,404.706546495746));
#48886=CARTESIAN_POINT('',(350.793381459681,-210.47200726879,386.345586463583));
#48887=CARTESIAN_POINT('Origin',(347.290676030261,-210.47200726879,389.91364681547));
#48888=CARTESIAN_POINT('',(341.995805744459,-210.47200726879,377.709152887802));
#48889=CARTESIAN_POINT('',(349.71557428276,-210.47200726879,385.287521106456));
#48890=CARTESIAN_POINT('Origin',(375.115917770964,-210.47200726879,445.000000551892));
#48891=CARTESIAN_POINT('Origin',(375.115917770964,-210.47200726879,445.000000551892));
#48892=CARTESIAN_POINT('Origin',(375.115917770964,-210.47200726879,445.000000551892));
#48893=CARTESIAN_POINT('Origin',(375.115917770964,-195.47200726879,445.000000551892));
#48894=CARTESIAN_POINT('Origin',(438.073398571173,-210.47200726879,453.263273266005));
#48895=CARTESIAN_POINT('',(449.951557303508,-195.47200726879,449.962565992797));
#48896=CARTESIAN_POINT('',(449.951557303507,-210.47200726879,449.962565992797));
#48897=CARTESIAN_POINT('',(438.073398571173,-195.47200726879,453.263273266005));
#48898=CARTESIAN_POINT('',(438.073398571173,-210.47200726879,453.263273266005));
#48899=CARTESIAN_POINT('',(390.584364046299,-195.47200726879,466.459544269457));
#48900=CARTESIAN_POINT('Origin',(436.734720378913,-210.47200726879,448.44581120621));
#48901=CARTESIAN_POINT('',(431.749931923224,-195.47200726879,448.056088160926));
#48902=CARTESIAN_POINT('',(431.749931923224,-210.47200726879,448.056088160926));
#48903=CARTESIAN_POINT('Origin',(436.734720378913,-195.47200726879,448.44581120621));
#48904=CARTESIAN_POINT('Origin',(433.14196495934,-210.47200726879,430.251161579503));
#48905=CARTESIAN_POINT('',(433.14196495934,-195.47200726879,430.251161579503));
#48906=CARTESIAN_POINT('',(433.14196495934,-210.47200726879,430.251161579503));
#48907=CARTESIAN_POINT('',(433.608541542394,-195.47200726879,424.283370880314));
#48908=CARTESIAN_POINT('Origin',(420.176185455833,-210.47200726879,383.591590074578));
#48909=CARTESIAN_POINT('',(420.687969084835,-195.47200726879,385.433330852756));
#48910=CARTESIAN_POINT('',(420.687969084835,-210.47200726879,385.433330852756));
#48911=CARTESIAN_POINT('',(420.081814582884,-195.47200726879,383.251980374046));
#48912=CARTESIAN_POINT('Origin',(336.480973282039,-210.47200726879,495.391141926086));
#48913=CARTESIAN_POINT('',(333.400390264926,-195.47200726879,507.328282775076));
#48914=CARTESIAN_POINT('',(333.400390264926,-210.47200726879,507.328282775076));
#48915=CARTESIAN_POINT('',(336.480973282039,-195.47200726879,495.391141926086));
#48916=CARTESIAN_POINT('',(336.480973282039,-210.47200726879,495.391141926086));
#48917=CARTESIAN_POINT('',(346.449185288851,-195.47200726879,456.764703334135));
#48918=CARTESIAN_POINT('Origin',(341.322356903719,-210.47200726879,496.640543633995));
#48919=CARTESIAN_POINT('',(344.15226118922,-195.47200726879,492.518451721519));
#48920=CARTESIAN_POINT('',(344.15226118922,-210.47200726879,492.518451721519));
#48921=CARTESIAN_POINT('Origin',(341.322356903719,-195.47200726879,496.640543633995));
#48922=CARTESIAN_POINT('Origin',(358.875763403191,-210.47200726879,502.626450984414));
#48923=CARTESIAN_POINT('',(358.875763403191,-195.47200726879,502.626450984414));
#48924=CARTESIAN_POINT('',(358.875763403191,-210.47200726879,502.626450984414));
#48925=CARTESIAN_POINT('',(325.221168140732,-195.47200726879,479.521851333988));
#48926=CARTESIAN_POINT('Origin',(405.767027407906,-210.47200726879,514.727542306972));
#48927=CARTESIAN_POINT('',(403.916141292317,-195.47200726879,514.24988954184));
#48928=CARTESIAN_POINT('',(403.916141292317,-210.47200726879,514.24988954184));
#48929=CARTESIAN_POINT('',(354.564704687327,-195.47200726879,501.513908673498));
#48930=CARTESIAN_POINT('Origin',(375.115917770964,-210.47200726879,445.000000551892));
#48931=CARTESIAN_POINT('',(300.743642935741,-195.47200726879,435.316781261079));
#48932=CARTESIAN_POINT('Origin',(375.115917770964,-195.47200726879,445.000000551892));
#48933=CARTESIAN_POINT('',(300.743642935741,-210.47200726879,435.316781261079));
#48934=CARTESIAN_POINT('Origin',(375.115917770964,-210.47200726879,445.000000551892));
#48935=CARTESIAN_POINT('Origin',(375.115917770964,-195.47200726879,445.000000551892));
#48936=CARTESIAN_POINT('Origin',(347.290676030261,-210.47200726879,389.91364681547));
#48937=CARTESIAN_POINT('',(349.445560200449,-195.47200726879,394.42546177323));
#48938=CARTESIAN_POINT('',(349.445560200449,-210.47200726879,394.42546177323));
#48939=CARTESIAN_POINT('',(350.793381459681,-195.47200726879,386.345586463583));
#48940=CARTESIAN_POINT('Origin',(347.290676030261,-195.47200726879,389.91364681547));
#48941=CARTESIAN_POINT('',(350.793381459681,-210.47200726879,386.345586463583));
#48942=CARTESIAN_POINT('Origin',(333.330024950362,-210.47200726879,402.122389091758));
#48943=CARTESIAN_POINT('',(333.330024950362,-195.47200726879,402.122389091758));
#48944=CARTESIAN_POINT('',(333.330024950362,-210.47200726879,402.122389091758));
#48945=CARTESIAN_POINT('',(327.919413934783,-195.47200726879,404.706546495746));
#48946=CARTESIAN_POINT('Origin',(299.404540449154,-210.47200726879,436.680869274125));
#48947=CARTESIAN_POINT('',(312.102604347699,-195.47200726879,423.745879662505));
#48948=CARTESIAN_POINT('Origin',(350.793381459681,-210.47200726879,386.345586463583));
#48949=CARTESIAN_POINT('',(341.995805744459,-195.47200726879,377.709152887802));
#48950=CARTESIAN_POINT('',(341.995805744459,-210.47200726879,377.709152887802));
#48951=CARTESIAN_POINT('',(349.71557428276,-195.47200726879,385.287521106456));
#48952=CARTESIAN_POINT('Origin',(375.115917770964,-210.47200726879,445.000000551892));
#48953=CARTESIAN_POINT('Origin',(375.115917770964,-195.47200726879,445.000000551892));
#48954=CARTESIAN_POINT('Origin',(323.651078177653,-195.47200726879,409.682356624389));
#61751=UNCERTAINTY_MEASURE_WITH_UNIT(LENGTH_MEASURE(0.01),#61812,
'DISTANCE_ACCURACY_VALUE',
'Maximum model space distance between geometric entities at asserted c
onnectivities');
#61780=UNCERTAINTY_MEASURE_WITH_UNIT(LENGTH_MEASURE(0.01),#61812,
'DISTANCE_ACCURACY_VALUE',
'Maximum model space distance between geometric entities at asserted c
onnectivities');
#61782=(
GEOMETRIC_REPRESENTATION_CONTEXT(3)
GLOBAL_UNCERTAINTY_ASSIGNED_CONTEXT((#61751))
GLOBAL_UNIT_ASSIGNED_CONTEXT((#61812,#61814,#61815))
REPRESENTATION_CONTEXT('','3D')
);
#61811=(
GEOMETRIC_REPRESENTATION_CONTEXT(3)
GLOBAL_UNCERTAINTY_ASSIGNED_CONTEXT((#61780))
GLOBAL_UNIT_ASSIGNED_CONTEXT((#61812,#61814,#61815))
REPRESENTATION_CONTEXT('','3D')
);
#61812=(
LENGTH_UNIT()
NAMED_UNIT(*)
SI_UNIT(.MILLI.,.METRE.)
);
#61814=(
NAMED_UNIT(*)
PLANE_ANGLE_UNIT()
SI_UNIT($,.RADIAN.)
);
#61815=(
NAMED_UNIT(*)
SI_UNIT($,.STERADIAN.)
SOLID_ANGLE_UNIT()
);
#61817=SHAPE_DEFINITION_REPRESENTATION(#61847,#61969);
#61847=PRODUCT_DEFINITION_SHAPE('',$,#62000);
#61969=SHAPE_REPRESENTATION('',(#34117),#61782);
#61998=PRODUCT_DEFINITION_CONTEXT('part definition',#62090,'design');
#62000=PRODUCT_DEFINITION('Shredder Cutting Blades',
'Shredder Cutting Blades',#62030,#61998);
#62030=PRODUCT_DEFINITION_FORMATION('',$,#62093);
#62090=APPLICATION_CONTEXT('Managed model based 3d engineering');
#62091=PRODUCT_CONTEXT('part definition',#62090,'mechanical');
#62093=PRODUCT('Shredder Cutting Blades','Shredder Cutting Blades',$,(#62091));
#62143=COLOUR_RGB('Sky Blue',0.24,0.69,0.87);
#62144=FILL_AREA_STYLE_COLOUR('',#62143);
#62145=FILL_AREA_STYLE('',(#62144));
#62146=SURFACE_STYLE_FILL_AREA(#62145);
#62147=SURFACE_SIDE_STYLE('',(#62146));
#62148=SURFACE_STYLE_USAGE(.BOTH.,#62147);
#62149=PRESENTATION_STYLE_ASSIGNMENT((#62148));
ENDSEC;
END-ISO-10303-21;
